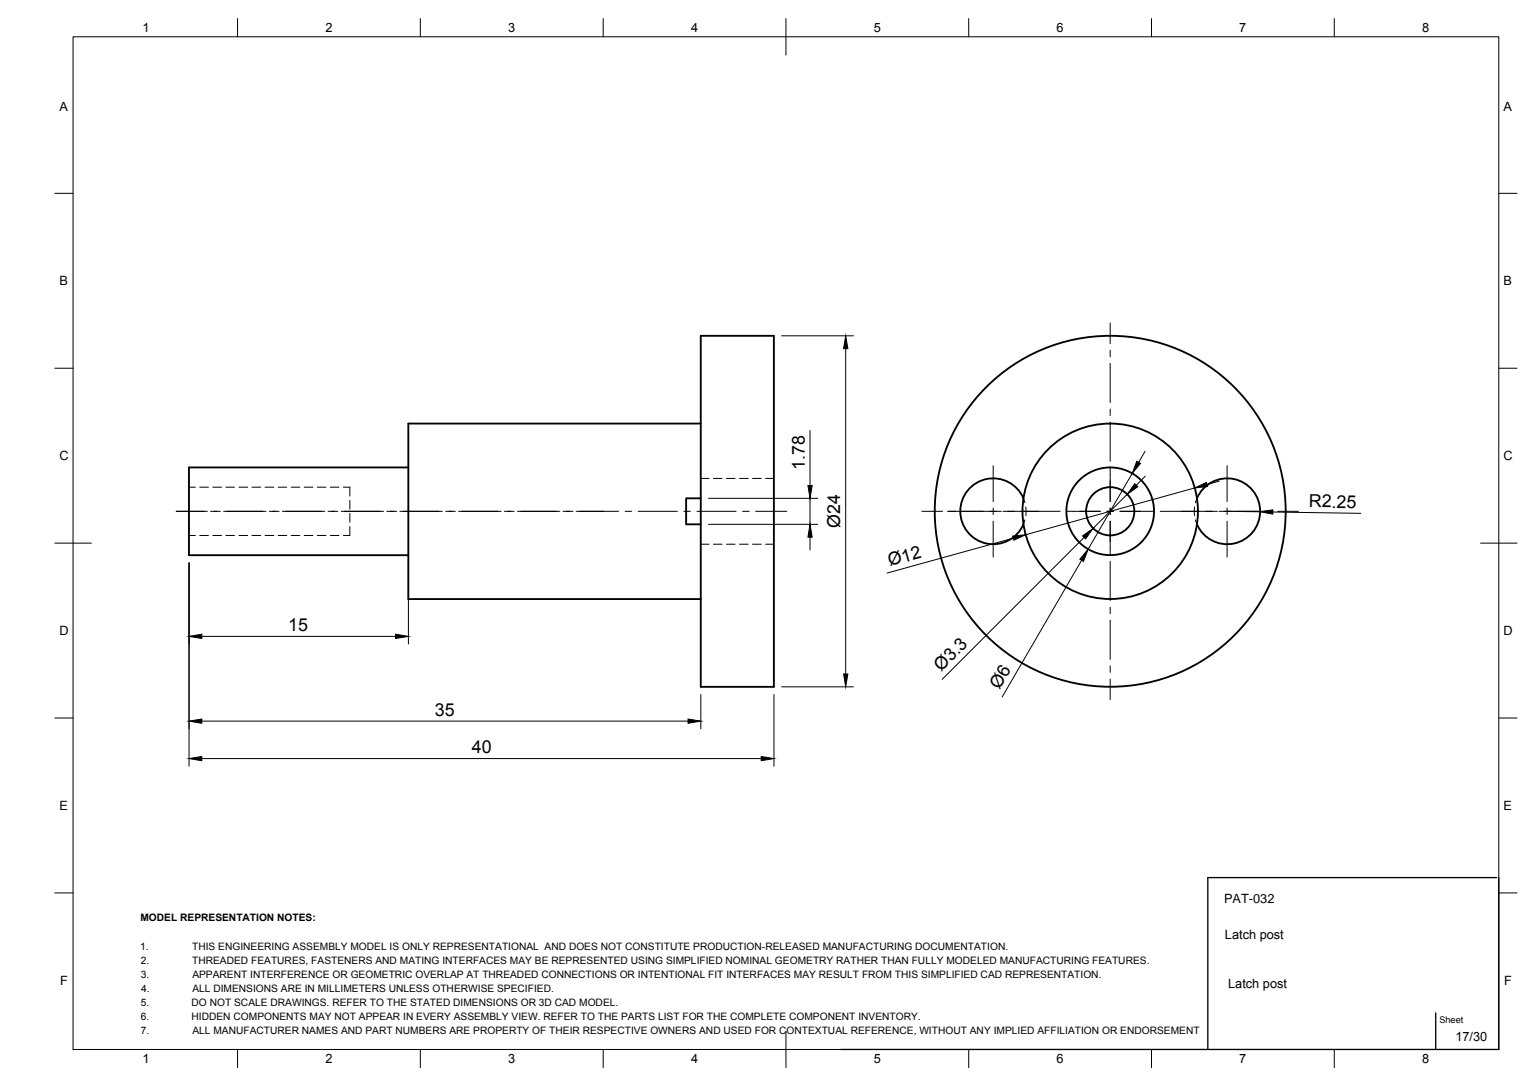
ISO-10303-21;
HEADER;
/* Generated by software containing ST-Developer
 * from STEP Tools, Inc. (www.steptools.com) 
 */

FILE_DESCRIPTION(
/* description */ ('Drill jig with bushing plate'),
/* implementation_level */ '2;1');

FILE_NAME(
/* name */ 'Latch post.step',
/* time_stamp */ '2026-10-27T10:51:08-07:00',
/* author */ (''),
/* organization */ (''),
/* preprocessor_version */ 'ST-DEVELOPER v20.2',
/* originating_system */ 'Autodesk Translation Framework v15.17.0.0',
/* authorisation */ '');

FILE_SCHEMA (('AUTOMOTIVE_DESIGN { 1 0 10303 214 3 1 1 }'));
ENDSEC;

DATA;
#10=MECHANICAL_DESIGN_GEOMETRIC_PRESENTATION_REPRESENTATION('',(#235),#6638);
#187=SHAPE_REPRESENTATION_RELATIONSHIP('SRR','None',#6751,#211);
#211=ADVANCED_BREP_SHAPE_REPRESENTATION('',(#259),#6624);
#235=STYLED_ITEM('',(#6957),#259);
#259=MANIFOLD_SOLID_BREP('Body1',#3602);
#334=FACE_BOUND('',#890,.T.);
#335=FACE_BOUND('',#894,.T.);
#336=FACE_BOUND('',#896,.T.);
#337=FACE_BOUND('',#898,.T.);
#338=FACE_BOUND('',#899,.T.);
#431=PLANE('',#4083);
#432=PLANE('',#4084);
#433=PLANE('',#4091);
#434=PLANE('',#4103);
#435=PLANE('',#4110);
#436=PLANE('',#4111);
#437=PLANE('',#4112);
#603=FACE_OUTER_BOUND('',#882,.T.);
#604=FACE_OUTER_BOUND('',#883,.T.);
#605=FACE_OUTER_BOUND('',#884,.T.);
#606=FACE_OUTER_BOUND('',#885,.T.);
#607=FACE_OUTER_BOUND('',#886,.T.);
#608=FACE_OUTER_BOUND('',#887,.T.);
#609=FACE_OUTER_BOUND('',#888,.T.);
#610=FACE_OUTER_BOUND('',#889,.T.);
#611=FACE_OUTER_BOUND('',#891,.T.);
#612=FACE_OUTER_BOUND('',#892,.T.);
#613=FACE_OUTER_BOUND('',#893,.T.);
#614=FACE_OUTER_BOUND('',#895,.T.);
#615=FACE_OUTER_BOUND('',#897,.T.);
#882=EDGE_LOOP('',(#2855,#2856,#2857,#2858));
#883=EDGE_LOOP('',(#2859));
#884=EDGE_LOOP('',(#2860,#2861));
#885=EDGE_LOOP('',(#2862,#2863,#2864,#2865,#2866,#2867,#2868,#2869));
#886=EDGE_LOOP('',(#2870,#2871));
#887=EDGE_LOOP('',(#2872,#2873,#2874,#2875,#2876,#2877,#2878,#2879));
#888=EDGE_LOOP('',(#2880,#2881,#2882,#2883,#2884,#2885,#2886,#2887,#2888,
#2889,#2890,#2891));
#889=EDGE_LOOP('',(#2892));
#890=EDGE_LOOP('',(#2893,#2894,#2895,#2896,#2897,#2898,#2899));
#891=EDGE_LOOP('',(#2900,#2901,#2902,#2903));
#892=EDGE_LOOP('',(#2904,#2905,#2906,#2907));
#893=EDGE_LOOP('',(#2908));
#894=EDGE_LOOP('',(#2909));
#895=EDGE_LOOP('',(#2910));
#896=EDGE_LOOP('',(#2911));
#897=EDGE_LOOP('',(#2912));
#898=EDGE_LOOP('',(#2913));
#899=EDGE_LOOP('',(#2914));
#1155=LINE('',#6054,#1416);
#1156=LINE('',#6066,#1417);
#1157=LINE('',#6069,#1418);
#1158=LINE('',#6071,#1419);
#1159=LINE('',#6082,#1420);
#1160=LINE('',#6085,#1421);
#1161=LINE('',#6087,#1422);
#1162=LINE('',#6093,#1423);
#1163=LINE('',#6102,#1424);
#1164=LINE('',#6108,#1425);
#1416=VECTOR('',#4856,0.164999999999999);
#1417=VECTOR('',#4871,0.225);
#1418=VECTOR('',#4874,1.);
#1419=VECTOR('',#4875,1.);
#1420=VECTOR('',#4888,0.225);
#1421=VECTOR('',#4891,1.);
#1422=VECTOR('',#4892,1.);
#1423=VECTOR('',#4899,0.6);
#1424=VECTOR('',#4912,1.2);
#1425=VECTOR('',#4919,0.300000000000001);
#1634=CIRCLE('',#4081,0.164999999999999);
#1635=CIRCLE('',#4082,0.164999999999999);
#1636=CIRCLE('',#4085,0.6);
#1637=CIRCLE('',#4086,0.225);
#1638=CIRCLE('',#4088,0.225);
#1639=CIRCLE('',#4089,0.225);
#1640=CIRCLE('',#4090,0.225);
#1641=CIRCLE('',#4092,0.6);
#1642=CIRCLE('',#4093,0.225);
#1643=CIRCLE('',#4095,0.225);
#1644=CIRCLE('',#4096,0.225);
#1645=CIRCLE('',#4097,0.225);
#1646=CIRCLE('',#4099,0.6);
#1647=CIRCLE('',#4100,0.6);
#1648=CIRCLE('',#4101,0.6);
#1649=CIRCLE('',#4102,0.6);
#1650=CIRCLE('',#4104,1.2);
#1651=CIRCLE('',#4106,1.2);
#1652=CIRCLE('',#4108,0.300000000000001);
#1653=CIRCLE('',#4109,0.300000000000001);
#1860=VERTEX_POINT('',#6051);
#1861=VERTEX_POINT('',#6053);
#1862=VERTEX_POINT('',#6058);
#1863=VERTEX_POINT('',#6059);
#1864=VERTEX_POINT('',#6063);
#1865=VERTEX_POINT('',#6065);
#1866=VERTEX_POINT('',#6067);
#1867=VERTEX_POINT('',#6070);
#1868=VERTEX_POINT('',#6074);
#1869=VERTEX_POINT('',#6075);
#1870=VERTEX_POINT('',#6079);
#1871=VERTEX_POINT('',#6081);
#1872=VERTEX_POINT('',#6083);
#1873=VERTEX_POINT('',#6086);
#1874=VERTEX_POINT('',#6090);
#1875=VERTEX_POINT('',#6092);
#1876=VERTEX_POINT('',#6098);
#1877=VERTEX_POINT('',#6101);
#1878=VERTEX_POINT('',#6105);
#1879=VERTEX_POINT('',#6107);
#2215=EDGE_CURVE('',#1860,#1860,#1634,.T.);
#2216=EDGE_CURVE('',#1860,#1861,#1155,.T.);
#2217=EDGE_CURVE('',#1861,#1861,#1635,.T.);
#2218=EDGE_CURVE('',#1862,#1863,#1636,.T.);
#2219=EDGE_CURVE('',#1863,#1862,#1637,.T.);
#2220=EDGE_CURVE('',#1864,#1864,#1638,.T.);
#2221=EDGE_CURVE('',#1864,#1865,#1156,.T.);
#2222=EDGE_CURVE('',#1866,#1865,#1639,.T.);
#2223=EDGE_CURVE('',#1863,#1866,#1157,.T.);
#2224=EDGE_CURVE('',#1867,#1862,#1158,.T.);
#2225=EDGE_CURVE('',#1865,#1867,#1640,.T.);
#2226=EDGE_CURVE('',#1868,#1869,#1641,.T.);
#2227=EDGE_CURVE('',#1869,#1868,#1642,.T.);
#2228=EDGE_CURVE('',#1870,#1870,#1643,.T.);
#2229=EDGE_CURVE('',#1870,#1871,#1159,.T.);
#2230=EDGE_CURVE('',#1872,#1871,#1644,.T.);
#2231=EDGE_CURVE('',#1869,#1872,#1160,.T.);
#2232=EDGE_CURVE('',#1873,#1868,#1161,.T.);
#2233=EDGE_CURVE('',#1871,#1873,#1645,.T.);
#2234=EDGE_CURVE('',#1874,#1874,#1646,.T.);
#2235=EDGE_CURVE('',#1874,#1875,#1162,.T.);
#2236=EDGE_CURVE('',#1875,#1867,#1647,.T.);
#2237=EDGE_CURVE('',#1866,#1873,#1648,.T.);
#2238=EDGE_CURVE('',#1872,#1875,#1649,.T.);
#2239=EDGE_CURVE('',#1876,#1876,#1650,.T.);
#2240=EDGE_CURVE('',#1876,#1877,#1163,.T.);
#2241=EDGE_CURVE('',#1877,#1877,#1651,.T.);
#2242=EDGE_CURVE('',#1878,#1878,#1652,.T.);
#2243=EDGE_CURVE('',#1878,#1879,#1164,.T.);
#2244=EDGE_CURVE('',#1879,#1879,#1653,.T.);
#2855=ORIENTED_EDGE('',*,*,#2215,.F.);
#2856=ORIENTED_EDGE('',*,*,#2216,.T.);
#2857=ORIENTED_EDGE('',*,*,#2217,.F.);
#2858=ORIENTED_EDGE('',*,*,#2216,.F.);
#2859=ORIENTED_EDGE('',*,*,#2215,.T.);
#2860=ORIENTED_EDGE('',*,*,#2218,.F.);
#2861=ORIENTED_EDGE('',*,*,#2219,.F.);
#2862=ORIENTED_EDGE('',*,*,#2220,.F.);
#2863=ORIENTED_EDGE('',*,*,#2221,.T.);
#2864=ORIENTED_EDGE('',*,*,#2222,.F.);
#2865=ORIENTED_EDGE('',*,*,#2223,.F.);
#2866=ORIENTED_EDGE('',*,*,#2219,.T.);
#2867=ORIENTED_EDGE('',*,*,#2224,.F.);
#2868=ORIENTED_EDGE('',*,*,#2225,.F.);
#2869=ORIENTED_EDGE('',*,*,#2221,.F.);
#2870=ORIENTED_EDGE('',*,*,#2226,.F.);
#2871=ORIENTED_EDGE('',*,*,#2227,.F.);
#2872=ORIENTED_EDGE('',*,*,#2228,.F.);
#2873=ORIENTED_EDGE('',*,*,#2229,.T.);
#2874=ORIENTED_EDGE('',*,*,#2230,.F.);
#2875=ORIENTED_EDGE('',*,*,#2231,.F.);
#2876=ORIENTED_EDGE('',*,*,#2227,.T.);
#2877=ORIENTED_EDGE('',*,*,#2232,.F.);
#2878=ORIENTED_EDGE('',*,*,#2233,.F.);
#2879=ORIENTED_EDGE('',*,*,#2229,.F.);
#2880=ORIENTED_EDGE('',*,*,#2234,.F.);
#2881=ORIENTED_EDGE('',*,*,#2235,.T.);
#2882=ORIENTED_EDGE('',*,*,#2236,.T.);
#2883=ORIENTED_EDGE('',*,*,#2224,.T.);
#2884=ORIENTED_EDGE('',*,*,#2218,.T.);
#2885=ORIENTED_EDGE('',*,*,#2223,.T.);
#2886=ORIENTED_EDGE('',*,*,#2237,.T.);
#2887=ORIENTED_EDGE('',*,*,#2232,.T.);
#2888=ORIENTED_EDGE('',*,*,#2226,.T.);
#2889=ORIENTED_EDGE('',*,*,#2231,.T.);
#2890=ORIENTED_EDGE('',*,*,#2238,.T.);
#2891=ORIENTED_EDGE('',*,*,#2235,.F.);
#2892=ORIENTED_EDGE('',*,*,#2239,.T.);
#2893=ORIENTED_EDGE('',*,*,#2222,.T.);
#2894=ORIENTED_EDGE('',*,*,#2225,.T.);
#2895=ORIENTED_EDGE('',*,*,#2236,.F.);
#2896=ORIENTED_EDGE('',*,*,#2238,.F.);
#2897=ORIENTED_EDGE('',*,*,#2230,.T.);
#2898=ORIENTED_EDGE('',*,*,#2233,.T.);
#2899=ORIENTED_EDGE('',*,*,#2237,.F.);
#2900=ORIENTED_EDGE('',*,*,#2239,.F.);
#2901=ORIENTED_EDGE('',*,*,#2240,.T.);
#2902=ORIENTED_EDGE('',*,*,#2241,.T.);
#2903=ORIENTED_EDGE('',*,*,#2240,.F.);
#2904=ORIENTED_EDGE('',*,*,#2242,.F.);
#2905=ORIENTED_EDGE('',*,*,#2243,.T.);
#2906=ORIENTED_EDGE('',*,*,#2244,.F.);
#2907=ORIENTED_EDGE('',*,*,#2243,.F.);
#2908=ORIENTED_EDGE('',*,*,#2242,.T.);
#2909=ORIENTED_EDGE('',*,*,#2217,.T.);
#2910=ORIENTED_EDGE('',*,*,#2234,.T.);
#2911=ORIENTED_EDGE('',*,*,#2244,.T.);
#2912=ORIENTED_EDGE('',*,*,#2241,.F.);
#2913=ORIENTED_EDGE('',*,*,#2220,.T.);
#2914=ORIENTED_EDGE('',*,*,#2228,.T.);
#3340=CYLINDRICAL_SURFACE('',#4080,0.164999999999999);
#3341=CYLINDRICAL_SURFACE('',#4087,0.225);
#3342=CYLINDRICAL_SURFACE('',#4094,0.225);
#3343=CYLINDRICAL_SURFACE('',#4098,0.6);
#3344=CYLINDRICAL_SURFACE('',#4105,1.2);
#3345=CYLINDRICAL_SURFACE('',#4107,0.300000000000001);
#3478=ADVANCED_FACE('',(#603),#3340,.F.);
#3479=ADVANCED_FACE('',(#604),#431,.T.);
#3480=ADVANCED_FACE('',(#605),#432,.F.);
#3481=ADVANCED_FACE('',(#606),#3341,.F.);
#3482=ADVANCED_FACE('',(#607),#433,.F.);
#3483=ADVANCED_FACE('',(#608),#3342,.F.);
#3484=ADVANCED_FACE('',(#609),#3343,.T.);
#3485=ADVANCED_FACE('',(#610,#334),#434,.T.);
#3486=ADVANCED_FACE('',(#611),#3344,.T.);
#3487=ADVANCED_FACE('',(#612),#3345,.T.);
#3488=ADVANCED_FACE('',(#613,#335),#435,.T.);
#3489=ADVANCED_FACE('',(#614,#336),#436,.T.);
#3490=ADVANCED_FACE('',(#615,#337,#338),#437,.F.);
#3602=CLOSED_SHELL('',(#3478,#3479,#3480,#3481,#3482,#3483,#3484,#3485,
#3486,#3487,#3488,#3489,#3490));
#4079=AXIS2_PLACEMENT_3D('',#6049,#4850,#4851);
#4080=AXIS2_PLACEMENT_3D('',#6050,#4852,#4853);
#4081=AXIS2_PLACEMENT_3D('',#6052,#4854,#4855);
#4082=AXIS2_PLACEMENT_3D('',#6055,#4857,#4858);
#4083=AXIS2_PLACEMENT_3D('',#6056,#4859,#4860);
#4084=AXIS2_PLACEMENT_3D('',#6057,#4861,#4862);
#4085=AXIS2_PLACEMENT_3D('',#6060,#4863,#4864);
#4086=AXIS2_PLACEMENT_3D('',#6061,#4865,#4866);
#4087=AXIS2_PLACEMENT_3D('',#6062,#4867,#4868);
#4088=AXIS2_PLACEMENT_3D('',#6064,#4869,#4870);
#4089=AXIS2_PLACEMENT_3D('',#6068,#4872,#4873);
#4090=AXIS2_PLACEMENT_3D('',#6072,#4876,#4877);
#4091=AXIS2_PLACEMENT_3D('',#6073,#4878,#4879);
#4092=AXIS2_PLACEMENT_3D('',#6076,#4880,#4881);
#4093=AXIS2_PLACEMENT_3D('',#6077,#4882,#4883);
#4094=AXIS2_PLACEMENT_3D('',#6078,#4884,#4885);
#4095=AXIS2_PLACEMENT_3D('',#6080,#4886,#4887);
#4096=AXIS2_PLACEMENT_3D('',#6084,#4889,#4890);
#4097=AXIS2_PLACEMENT_3D('',#6088,#4893,#4894);
#4098=AXIS2_PLACEMENT_3D('',#6089,#4895,#4896);
#4099=AXIS2_PLACEMENT_3D('',#6091,#4897,#4898);
#4100=AXIS2_PLACEMENT_3D('',#6094,#4900,#4901);
#4101=AXIS2_PLACEMENT_3D('',#6095,#4902,#4903);
#4102=AXIS2_PLACEMENT_3D('',#6096,#4904,#4905);
#4103=AXIS2_PLACEMENT_3D('',#6097,#4906,#4907);
#4104=AXIS2_PLACEMENT_3D('',#6099,#4908,#4909);
#4105=AXIS2_PLACEMENT_3D('',#6100,#4910,#4911);
#4106=AXIS2_PLACEMENT_3D('',#6103,#4913,#4914);
#4107=AXIS2_PLACEMENT_3D('',#6104,#4915,#4916);
#4108=AXIS2_PLACEMENT_3D('',#6106,#4917,#4918);
#4109=AXIS2_PLACEMENT_3D('',#6109,#4920,#4921);
#4110=AXIS2_PLACEMENT_3D('',#6110,#4922,#4923);
#4111=AXIS2_PLACEMENT_3D('',#6111,#4924,#4925);
#4112=AXIS2_PLACEMENT_3D('',#6112,#4926,#4927);
#4850=DIRECTION('axis',(0.,0.,1.));
#4851=DIRECTION('refdir',(1.,0.,0.));
#4852=DIRECTION('center_axis',(0.,0.,1.));
#4853=DIRECTION('ref_axis',(1.,0.,0.));
#4854=DIRECTION('center_axis',(0.,0.,1.));
#4855=DIRECTION('ref_axis',(1.,0.,0.));
#4856=DIRECTION('',(0.,0.,1.));
#4857=DIRECTION('center_axis',(0.,0.,-1.));
#4858=DIRECTION('ref_axis',(1.,0.,0.));
#4859=DIRECTION('center_axis',(0.,0.,1.));
#4860=DIRECTION('ref_axis',(1.,0.,0.));
#4861=DIRECTION('center_axis',(0.,0.,1.));
#4862=DIRECTION('ref_axis',(1.,0.,0.));
#4863=DIRECTION('center_axis',(0.,0.,1.));
#4864=DIRECTION('ref_axis',(1.,0.,0.));
#4865=DIRECTION('center_axis',(0.,0.,1.));
#4866=DIRECTION('ref_axis',(1.,0.,0.));
#4867=DIRECTION('center_axis',(0.,0.,1.));
#4868=DIRECTION('ref_axis',(1.,0.,0.));
#4869=DIRECTION('center_axis',(0.,0.,1.));
#4870=DIRECTION('ref_axis',(1.,0.,0.));
#4871=DIRECTION('',(0.,0.,1.));
#4872=DIRECTION('center_axis',(0.,0.,-1.));
#4873=DIRECTION('ref_axis',(1.,0.,0.));
#4874=DIRECTION('',(0.,0.,-1.));
#4875=DIRECTION('',(0.,0.,1.));
#4876=DIRECTION('center_axis',(0.,0.,-1.));
#4877=DIRECTION('ref_axis',(1.,0.,0.));
#4878=DIRECTION('center_axis',(0.,0.,1.));
#4879=DIRECTION('ref_axis',(1.,0.,0.));
#4880=DIRECTION('center_axis',(0.,0.,1.));
#4881=DIRECTION('ref_axis',(1.,0.,0.));
#4882=DIRECTION('center_axis',(0.,0.,1.));
#4883=DIRECTION('ref_axis',(1.,0.,0.));
#4884=DIRECTION('center_axis',(0.,0.,1.));
#4885=DIRECTION('ref_axis',(1.,0.,0.));
#4886=DIRECTION('center_axis',(0.,0.,1.));
#4887=DIRECTION('ref_axis',(1.,0.,0.));
#4888=DIRECTION('',(0.,0.,1.));
#4889=DIRECTION('center_axis',(0.,0.,-1.));
#4890=DIRECTION('ref_axis',(1.,0.,0.));
#4891=DIRECTION('',(0.,0.,-1.));
#4892=DIRECTION('',(0.,0.,1.));
#4893=DIRECTION('center_axis',(0.,0.,-1.));
#4894=DIRECTION('ref_axis',(1.,0.,0.));
#4895=DIRECTION('center_axis',(0.,0.,1.));
#4896=DIRECTION('ref_axis',(1.,0.,0.));
#4897=DIRECTION('center_axis',(0.,0.,1.));
#4898=DIRECTION('ref_axis',(1.,0.,0.));
#4899=DIRECTION('',(0.,0.,-1.));
#4900=DIRECTION('center_axis',(0.,0.,1.));
#4901=DIRECTION('ref_axis',(1.,0.,0.));
#4902=DIRECTION('center_axis',(0.,0.,1.));
#4903=DIRECTION('ref_axis',(1.,0.,0.));
#4904=DIRECTION('center_axis',(0.,0.,1.));
#4905=DIRECTION('ref_axis',(1.,0.,0.));
#4906=DIRECTION('center_axis',(0.,0.,1.));
#4907=DIRECTION('ref_axis',(1.,0.,0.));
#4908=DIRECTION('center_axis',(0.,0.,1.));
#4909=DIRECTION('ref_axis',(1.,0.,0.));
#4910=DIRECTION('center_axis',(0.,0.,1.));
#4911=DIRECTION('ref_axis',(1.,0.,0.));
#4912=DIRECTION('',(0.,0.,-1.));
#4913=DIRECTION('center_axis',(0.,0.,1.));
#4914=DIRECTION('ref_axis',(1.,0.,0.));
#4915=DIRECTION('center_axis',(0.,0.,1.));
#4916=DIRECTION('ref_axis',(1.,0.,0.));
#4917=DIRECTION('center_axis',(0.,0.,1.));
#4918=DIRECTION('ref_axis',(1.,0.,0.));
#4919=DIRECTION('',(0.,0.,-1.));
#4920=DIRECTION('center_axis',(0.,0.,-1.));
#4921=DIRECTION('ref_axis',(1.,0.,0.));
#4922=DIRECTION('center_axis',(0.,0.,1.));
#4923=DIRECTION('ref_axis',(1.,0.,0.));
#4924=DIRECTION('center_axis',(0.,0.,1.));
#4925=DIRECTION('ref_axis',(1.,0.,0.));
#4926=DIRECTION('center_axis',(0.,0.,1.));
#4927=DIRECTION('ref_axis',(1.,0.,0.));
#6049=CARTESIAN_POINT('',(0.,0.,0.));
#6050=CARTESIAN_POINT('Origin',(9.2,3.5,3.9));
#6051=CARTESIAN_POINT('',(9.035,3.5,3.9));
#6052=CARTESIAN_POINT('Origin',(9.2,3.5,3.9));
#6053=CARTESIAN_POINT('',(9.035,3.5,5.));
#6054=CARTESIAN_POINT('',(9.035,3.5,3.9));
#6055=CARTESIAN_POINT('Origin',(9.2,3.5,5.));
#6056=CARTESIAN_POINT('Origin',(9.2,3.5,3.9));
#6057=CARTESIAN_POINT('Origin',(9.2,2.7,1.6));
#6058=CARTESIAN_POINT('',(9.11097948495089,2.906640625,1.6));
#6059=CARTESIAN_POINT('',(9.28902051504911,2.906640625,1.6));
#6060=CARTESIAN_POINT('Origin',(9.2,3.5,1.6));
#6061=CARTESIAN_POINT('Origin',(9.2,2.7,1.6));
#6062=CARTESIAN_POINT('Origin',(9.2,2.7,0.9));
#6063=CARTESIAN_POINT('',(8.975,2.7,1.));
#6064=CARTESIAN_POINT('Origin',(9.2,2.7,1.));
#6065=CARTESIAN_POINT('',(8.975,2.7,1.5));
#6066=CARTESIAN_POINT('',(8.975,2.7,0.9));
#6067=CARTESIAN_POINT('',(9.28902051504911,2.906640625,1.5));
#6068=CARTESIAN_POINT('Origin',(9.2,2.7,1.5));
#6069=CARTESIAN_POINT('',(9.28902051504911,2.906640625,0.9));
#6070=CARTESIAN_POINT('',(9.11097948495089,2.906640625,1.5));
#6071=CARTESIAN_POINT('',(9.11097948495089,2.906640625,0.9));
#6072=CARTESIAN_POINT('Origin',(9.2,2.7,1.5));
#6073=CARTESIAN_POINT('Origin',(9.2,4.3,1.6));
#6074=CARTESIAN_POINT('',(9.28902051504911,4.093359375,1.6));
#6075=CARTESIAN_POINT('',(9.11097948495089,4.093359375,1.6));
#6076=CARTESIAN_POINT('Origin',(9.2,3.5,1.6));
#6077=CARTESIAN_POINT('Origin',(9.2,4.3,1.6));
#6078=CARTESIAN_POINT('Origin',(9.2,4.3,0.9));
#6079=CARTESIAN_POINT('',(8.975,4.3,1.));
#6080=CARTESIAN_POINT('Origin',(9.2,4.3,1.));
#6081=CARTESIAN_POINT('',(8.975,4.3,1.5));
#6082=CARTESIAN_POINT('',(8.975,4.3,0.9));
#6083=CARTESIAN_POINT('',(9.11097948495089,4.093359375,1.5));
#6084=CARTESIAN_POINT('Origin',(9.2,4.3,1.5));
#6085=CARTESIAN_POINT('',(9.11097948495089,4.093359375,0.9));
#6086=CARTESIAN_POINT('',(9.28902051504911,4.093359375,1.5));
#6087=CARTESIAN_POINT('',(9.28902051504911,4.093359375,0.9));
#6088=CARTESIAN_POINT('Origin',(9.2,4.3,1.5));
#6089=CARTESIAN_POINT('Origin',(9.2,3.5,1.));
#6090=CARTESIAN_POINT('',(8.6,3.5,3.5));
#6091=CARTESIAN_POINT('Origin',(9.2,3.5,3.5));
#6092=CARTESIAN_POINT('',(8.6,3.5,1.5));
#6093=CARTESIAN_POINT('',(8.6,3.5,1.));
#6094=CARTESIAN_POINT('Origin',(9.2,3.5,1.5));
#6095=CARTESIAN_POINT('Origin',(9.2,3.5,1.5));
#6096=CARTESIAN_POINT('Origin',(9.2,3.5,1.5));
#6097=CARTESIAN_POINT('Origin',(9.2,3.5,1.5));
#6098=CARTESIAN_POINT('',(8.,3.5,1.5));
#6099=CARTESIAN_POINT('Origin',(9.2,3.5,1.5));
#6100=CARTESIAN_POINT('Origin',(9.2,3.5,1.));
#6101=CARTESIAN_POINT('',(8.,3.5,1.));
#6102=CARTESIAN_POINT('',(8.,3.5,1.));
#6103=CARTESIAN_POINT('Origin',(9.2,3.5,1.));
#6104=CARTESIAN_POINT('Origin',(9.2,3.5,3.5));
#6105=CARTESIAN_POINT('',(8.9,3.5,5.));
#6106=CARTESIAN_POINT('Origin',(9.2,3.5,5.));
#6107=CARTESIAN_POINT('',(8.9,3.5,3.5));
#6108=CARTESIAN_POINT('',(8.9,3.5,3.5));
#6109=CARTESIAN_POINT('Origin',(9.2,3.5,3.5));
#6110=CARTESIAN_POINT('Origin',(9.2,3.5,5.));
#6111=CARTESIAN_POINT('Origin',(9.2,3.5,3.5));
#6112=CARTESIAN_POINT('Origin',(9.2,3.5,1.));
#6595=UNCERTAINTY_MEASURE_WITH_UNIT(LENGTH_MEASURE(0.001),#6639,
'DISTANCE_ACCURACY_VALUE',
'Maximum model space distance between geometric entities at asserted c
onnectivities');
#6609=UNCERTAINTY_MEASURE_WITH_UNIT(LENGTH_MEASURE(0.001),#6639,
'DISTANCE_ACCURACY_VALUE',
'Maximum model space distance between geometric entities at asserted c
onnectivities');
#6624=(
GEOMETRIC_REPRESENTATION_CONTEXT(3)
GLOBAL_UNCERTAINTY_ASSIGNED_CONTEXT((#6595))
GLOBAL_UNIT_ASSIGNED_CONTEXT((#6639,#6641,#6642))
REPRESENTATION_CONTEXT('','3D')
);
#6638=(
GEOMETRIC_REPRESENTATION_CONTEXT(3)
GLOBAL_UNCERTAINTY_ASSIGNED_CONTEXT((#6609))
GLOBAL_UNIT_ASSIGNED_CONTEXT((#6639,#6641,#6642))
REPRESENTATION_CONTEXT('','3D')
);
#6639=(
LENGTH_UNIT()
NAMED_UNIT(*)
SI_UNIT(.CENTI.,.METRE.)
);
#6641=(
NAMED_UNIT(*)
PLANE_ANGLE_UNIT()
SI_UNIT($,.RADIAN.)
);
#6642=(
NAMED_UNIT(*)
SI_UNIT($,.STERADIAN.)
SOLID_ANGLE_UNIT()
);
#6657=SHAPE_DEFINITION_REPRESENTATION(#6685,#6751);
#6685=PRODUCT_DEFINITION_SHAPE('',$,#6780);
#6751=SHAPE_REPRESENTATION('',(#4079),#6624);
#6765=PRODUCT_DEFINITION_CONTEXT('part definition',#6851,'design');
#6780=PRODUCT_DEFINITION('Latch post','Latch post',#6808,#6765);
#6808=PRODUCT_DEFINITION_FORMATION('',$,#6867);
#6851=APPLICATION_CONTEXT(
'Core Data for Automotive Mechanical Design Process');
#6852=PRODUCT_CONTEXT('part definition',#6851,'mechanical');
#6867=PRODUCT('Latch post','Latch post','Latch post',(#6852));
#6951=COLOUR_RGB('Off White',0.89,0.88,0.83);
#6952=FILL_AREA_STYLE_COLOUR('',#6951);
#6953=FILL_AREA_STYLE('',(#6952));
#6954=SURFACE_STYLE_FILL_AREA(#6953);
#6955=SURFACE_SIDE_STYLE('',(#6954));
#6956=SURFACE_STYLE_USAGE(.BOTH.,#6955);
#6957=PRESENTATION_STYLE_ASSIGNMENT((#6956));
ENDSEC;
END-ISO-10303-21;
